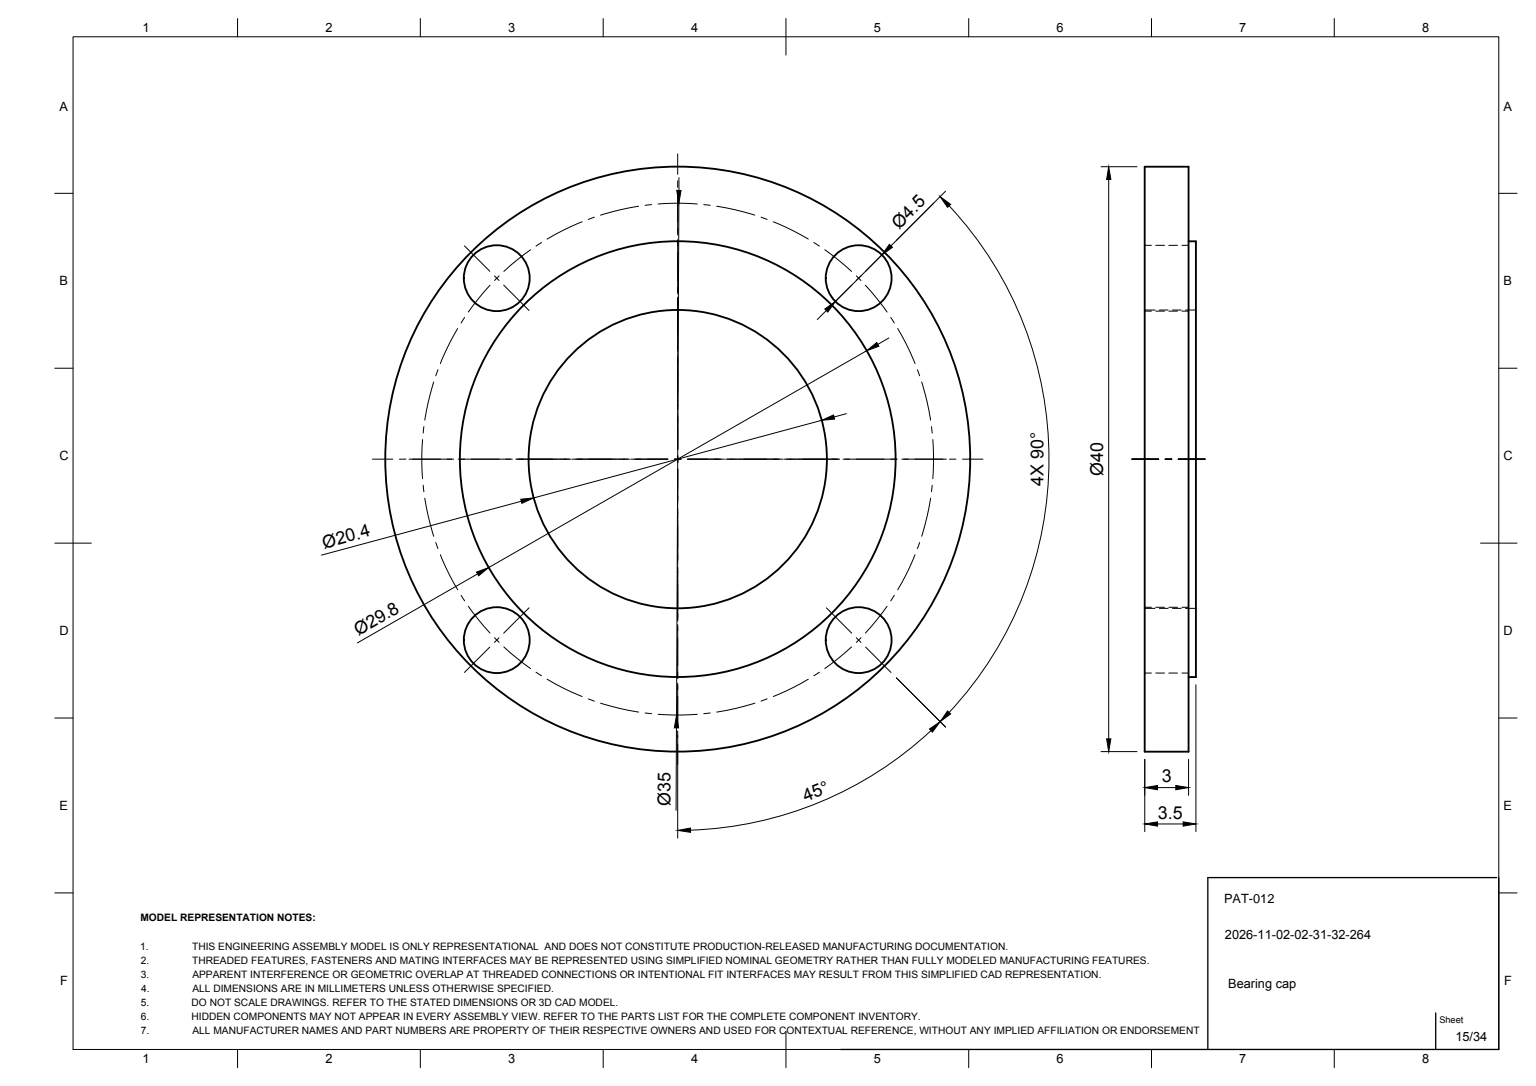
ISO-10303-21;
HEADER;
/* Generated by software containing ST-Developer
 * from STEP Tools, Inc. (www.steptools.com) 
 */

FILE_DESCRIPTION(
/* description */ ('Belt tensioner idler arm'),
/* implementation_level */ '2;1');

FILE_NAME(
/* name */ 'Bearing cap.step',
/* time_stamp */ '2026-10-28T03:22:15-07:00',
/* author */ (''),
/* organization */ (''),
/* preprocessor_version */ 'ST-DEVELOPER v20.2',
/* originating_system */ 'Autodesk Translation Framework v15.17.0.0',
/* authorisation */ '');

FILE_SCHEMA (('AUTOMOTIVE_DESIGN { 1 0 10303 214 3 1 1 }'));
ENDSEC;

DATA;
#10=MECHANICAL_DESIGN_GEOMETRIC_PRESENTATION_REPRESENTATION('',(#460),#12779);
#392=SHAPE_REPRESENTATION_RELATIONSHIP('SRR','None',#12939,#426);
#426=ADVANCED_BREP_SHAPE_REPRESENTATION('',(#500),#12756);
#460=STYLED_ITEM('',(#13184),#500);
#500=MANIFOLD_SOLID_BREP('Body1',#6196);
#582=FACE_BOUND('',#1400,.T.);
#583=FACE_BOUND('',#1404,.T.);
#584=FACE_BOUND('',#1405,.T.);
#585=FACE_BOUND('',#1406,.T.);
#586=FACE_BOUND('',#1407,.T.);
#587=FACE_BOUND('',#1408,.T.);
#588=FACE_BOUND('',#1410,.T.);
#589=FACE_BOUND('',#1411,.T.);
#590=FACE_BOUND('',#1412,.T.);
#591=FACE_BOUND('',#1413,.T.);
#592=FACE_BOUND('',#1414,.T.);
#744=PLANE('',#6866);
#745=PLANE('',#6873);
#746=PLANE('',#6874);
#972=FACE_OUTER_BOUND('',#1394,.T.);
#973=FACE_OUTER_BOUND('',#1395,.T.);
#974=FACE_OUTER_BOUND('',#1396,.T.);
#975=FACE_OUTER_BOUND('',#1397,.T.);
#976=FACE_OUTER_BOUND('',#1398,.T.);
#977=FACE_OUTER_BOUND('',#1399,.T.);
#978=FACE_OUTER_BOUND('',#1401,.T.);
#979=FACE_OUTER_BOUND('',#1402,.T.);
#980=FACE_OUTER_BOUND('',#1403,.T.);
#981=FACE_OUTER_BOUND('',#1409,.T.);
#1394=EDGE_LOOP('',(#4638,#4639,#4640,#4641));
#1395=EDGE_LOOP('',(#4642,#4643,#4644,#4645));
#1396=EDGE_LOOP('',(#4646,#4647,#4648,#4649));
#1397=EDGE_LOOP('',(#4650,#4651,#4652,#4653));
#1398=EDGE_LOOP('',(#4654,#4655,#4656,#4657));
#1399=EDGE_LOOP('',(#4658));
#1400=EDGE_LOOP('',(#4659));
#1401=EDGE_LOOP('',(#4660,#4661,#4662,#4663));
#1402=EDGE_LOOP('',(#4664,#4665,#4666,#4667));
#1403=EDGE_LOOP('',(#4668));
#1404=EDGE_LOOP('',(#4669));
#1405=EDGE_LOOP('',(#4670));
#1406=EDGE_LOOP('',(#4671));
#1407=EDGE_LOOP('',(#4672));
#1408=EDGE_LOOP('',(#4673));
#1409=EDGE_LOOP('',(#4674));
#1410=EDGE_LOOP('',(#4675));
#1411=EDGE_LOOP('',(#4676));
#1412=EDGE_LOOP('',(#4677));
#1413=EDGE_LOOP('',(#4678));
#1414=EDGE_LOOP('',(#4679));
#1861=LINE('',#10780,#2210);
#1862=LINE('',#10786,#2211);
#1863=LINE('',#10792,#2212);
#1864=LINE('',#10798,#2213);
#1865=LINE('',#10804,#2214);
#1866=LINE('',#10811,#2215);
#1867=LINE('',#10817,#2216);
#2210=VECTOR('',#8089,0.225);
#2211=VECTOR('',#8096,0.225);
#2212=VECTOR('',#8103,0.225);
#2213=VECTOR('',#8110,0.225);
#2214=VECTOR('',#8117,1.49);
#2215=VECTOR('',#8126,1.02);
#2216=VECTOR('',#8133,2.);
#2502=CIRCLE('',#6852,0.225);
#2503=CIRCLE('',#6853,0.225);
#2504=CIRCLE('',#6855,0.225);
#2505=CIRCLE('',#6856,0.225);
#2506=CIRCLE('',#6858,0.225);
#2507=CIRCLE('',#6859,0.225);
#2508=CIRCLE('',#6861,0.225);
#2509=CIRCLE('',#6862,0.225);
#2510=CIRCLE('',#6864,1.49);
#2511=CIRCLE('',#6865,1.49);
#2512=CIRCLE('',#6867,1.02);
#2513=CIRCLE('',#6869,1.02);
#2514=CIRCLE('',#6871,2.);
#2515=CIRCLE('',#6872,2.);
#2947=VERTEX_POINT('',#10777);
#2948=VERTEX_POINT('',#10779);
#2949=VERTEX_POINT('',#10783);
#2950=VERTEX_POINT('',#10785);
#2951=VERTEX_POINT('',#10789);
#2952=VERTEX_POINT('',#10791);
#2953=VERTEX_POINT('',#10795);
#2954=VERTEX_POINT('',#10797);
#2955=VERTEX_POINT('',#10801);
#2956=VERTEX_POINT('',#10803);
#2957=VERTEX_POINT('',#10807);
#2958=VERTEX_POINT('',#10810);
#2959=VERTEX_POINT('',#10814);
#2960=VERTEX_POINT('',#10816);
#3574=EDGE_CURVE('',#2947,#2947,#2502,.T.);
#3575=EDGE_CURVE('',#2947,#2948,#1861,.T.);
#3576=EDGE_CURVE('',#2948,#2948,#2503,.T.);
#3577=EDGE_CURVE('',#2949,#2949,#2504,.T.);
#3578=EDGE_CURVE('',#2949,#2950,#1862,.T.);
#3579=EDGE_CURVE('',#2950,#2950,#2505,.T.);
#3580=EDGE_CURVE('',#2951,#2951,#2506,.T.);
#3581=EDGE_CURVE('',#2951,#2952,#1863,.T.);
#3582=EDGE_CURVE('',#2952,#2952,#2507,.T.);
#3583=EDGE_CURVE('',#2953,#2953,#2508,.T.);
#3584=EDGE_CURVE('',#2953,#2954,#1864,.T.);
#3585=EDGE_CURVE('',#2954,#2954,#2509,.T.);
#3586=EDGE_CURVE('',#2955,#2955,#2510,.T.);
#3587=EDGE_CURVE('',#2955,#2956,#1865,.T.);
#3588=EDGE_CURVE('',#2956,#2956,#2511,.T.);
#3589=EDGE_CURVE('',#2957,#2957,#2512,.T.);
#3590=EDGE_CURVE('',#2957,#2958,#1866,.T.);
#3591=EDGE_CURVE('',#2958,#2958,#2513,.T.);
#3592=EDGE_CURVE('',#2959,#2959,#2514,.T.);
#3593=EDGE_CURVE('',#2959,#2960,#1867,.T.);
#3594=EDGE_CURVE('',#2960,#2960,#2515,.T.);
#4638=ORIENTED_EDGE('',*,*,#3574,.F.);
#4639=ORIENTED_EDGE('',*,*,#3575,.T.);
#4640=ORIENTED_EDGE('',*,*,#3576,.F.);
#4641=ORIENTED_EDGE('',*,*,#3575,.F.);
#4642=ORIENTED_EDGE('',*,*,#3577,.F.);
#4643=ORIENTED_EDGE('',*,*,#3578,.T.);
#4644=ORIENTED_EDGE('',*,*,#3579,.F.);
#4645=ORIENTED_EDGE('',*,*,#3578,.F.);
#4646=ORIENTED_EDGE('',*,*,#3580,.F.);
#4647=ORIENTED_EDGE('',*,*,#3581,.T.);
#4648=ORIENTED_EDGE('',*,*,#3582,.F.);
#4649=ORIENTED_EDGE('',*,*,#3581,.F.);
#4650=ORIENTED_EDGE('',*,*,#3583,.F.);
#4651=ORIENTED_EDGE('',*,*,#3584,.T.);
#4652=ORIENTED_EDGE('',*,*,#3585,.F.);
#4653=ORIENTED_EDGE('',*,*,#3584,.F.);
#4654=ORIENTED_EDGE('',*,*,#3586,.F.);
#4655=ORIENTED_EDGE('',*,*,#3587,.T.);
#4656=ORIENTED_EDGE('',*,*,#3588,.F.);
#4657=ORIENTED_EDGE('',*,*,#3587,.F.);
#4658=ORIENTED_EDGE('',*,*,#3586,.T.);
#4659=ORIENTED_EDGE('',*,*,#3589,.T.);
#4660=ORIENTED_EDGE('',*,*,#3589,.F.);
#4661=ORIENTED_EDGE('',*,*,#3590,.T.);
#4662=ORIENTED_EDGE('',*,*,#3591,.T.);
#4663=ORIENTED_EDGE('',*,*,#3590,.F.);
#4664=ORIENTED_EDGE('',*,*,#3592,.F.);
#4665=ORIENTED_EDGE('',*,*,#3593,.T.);
#4666=ORIENTED_EDGE('',*,*,#3594,.T.);
#4667=ORIENTED_EDGE('',*,*,#3593,.F.);
#4668=ORIENTED_EDGE('',*,*,#3592,.T.);
#4669=ORIENTED_EDGE('',*,*,#3588,.T.);
#4670=ORIENTED_EDGE('',*,*,#3585,.T.);
#4671=ORIENTED_EDGE('',*,*,#3582,.T.);
#4672=ORIENTED_EDGE('',*,*,#3579,.T.);
#4673=ORIENTED_EDGE('',*,*,#3576,.T.);
#4674=ORIENTED_EDGE('',*,*,#3594,.F.);
#4675=ORIENTED_EDGE('',*,*,#3591,.F.);
#4676=ORIENTED_EDGE('',*,*,#3583,.T.);
#4677=ORIENTED_EDGE('',*,*,#3580,.T.);
#4678=ORIENTED_EDGE('',*,*,#3577,.T.);
#4679=ORIENTED_EDGE('',*,*,#3574,.T.);
#5704=CYLINDRICAL_SURFACE('',#6851,0.225);
#5705=CYLINDRICAL_SURFACE('',#6854,0.225);
#5706=CYLINDRICAL_SURFACE('',#6857,0.225);
#5707=CYLINDRICAL_SURFACE('',#6860,0.225);
#5708=CYLINDRICAL_SURFACE('',#6863,1.49);
#5709=CYLINDRICAL_SURFACE('',#6868,1.02);
#5710=CYLINDRICAL_SURFACE('',#6870,2.);
#5949=ADVANCED_FACE('',(#972),#5704,.F.);
#5950=ADVANCED_FACE('',(#973),#5705,.F.);
#5951=ADVANCED_FACE('',(#974),#5706,.F.);
#5952=ADVANCED_FACE('',(#975),#5707,.F.);
#5953=ADVANCED_FACE('',(#976),#5708,.T.);
#5954=ADVANCED_FACE('',(#977,#582),#744,.T.);
#5955=ADVANCED_FACE('',(#978),#5709,.F.);
#5956=ADVANCED_FACE('',(#979),#5710,.T.);
#5957=ADVANCED_FACE('',(#980,#583,#584,#585,#586,#587),#745,.T.);
#5958=ADVANCED_FACE('',(#981,#588,#589,#590,#591,#592),#746,.F.);
#6196=CLOSED_SHELL('',(#5949,#5950,#5951,#5952,#5953,#5954,#5955,#5956,
#5957,#5958));
#6850=AXIS2_PLACEMENT_3D('',#10775,#8083,#8084);
#6851=AXIS2_PLACEMENT_3D('',#10776,#8085,#8086);
#6852=AXIS2_PLACEMENT_3D('',#10778,#8087,#8088);
#6853=AXIS2_PLACEMENT_3D('',#10781,#8090,#8091);
#6854=AXIS2_PLACEMENT_3D('',#10782,#8092,#8093);
#6855=AXIS2_PLACEMENT_3D('',#10784,#8094,#8095);
#6856=AXIS2_PLACEMENT_3D('',#10787,#8097,#8098);
#6857=AXIS2_PLACEMENT_3D('',#10788,#8099,#8100);
#6858=AXIS2_PLACEMENT_3D('',#10790,#8101,#8102);
#6859=AXIS2_PLACEMENT_3D('',#10793,#8104,#8105);
#6860=AXIS2_PLACEMENT_3D('',#10794,#8106,#8107);
#6861=AXIS2_PLACEMENT_3D('',#10796,#8108,#8109);
#6862=AXIS2_PLACEMENT_3D('',#10799,#8111,#8112);
#6863=AXIS2_PLACEMENT_3D('',#10800,#8113,#8114);
#6864=AXIS2_PLACEMENT_3D('',#10802,#8115,#8116);
#6865=AXIS2_PLACEMENT_3D('',#10805,#8118,#8119);
#6866=AXIS2_PLACEMENT_3D('',#10806,#8120,#8121);
#6867=AXIS2_PLACEMENT_3D('',#10808,#8122,#8123);
#6868=AXIS2_PLACEMENT_3D('',#10809,#8124,#8125);
#6869=AXIS2_PLACEMENT_3D('',#10812,#8127,#8128);
#6870=AXIS2_PLACEMENT_3D('',#10813,#8129,#8130);
#6871=AXIS2_PLACEMENT_3D('',#10815,#8131,#8132);
#6872=AXIS2_PLACEMENT_3D('',#10818,#8134,#8135);
#6873=AXIS2_PLACEMENT_3D('',#10819,#8136,#8137);
#6874=AXIS2_PLACEMENT_3D('',#10820,#8138,#8139);
#8083=DIRECTION('axis',(0.,0.,1.));
#8084=DIRECTION('refdir',(1.,0.,0.));
#8085=DIRECTION('center_axis',(0.,0.,1.));
#8086=DIRECTION('ref_axis',(1.,0.,0.));
#8087=DIRECTION('center_axis',(0.,0.,1.));
#8088=DIRECTION('ref_axis',(1.,0.,0.));
#8089=DIRECTION('',(0.,0.,1.));
#8090=DIRECTION('center_axis',(0.,0.,-1.));
#8091=DIRECTION('ref_axis',(1.,0.,0.));
#8092=DIRECTION('center_axis',(0.,0.,1.));
#8093=DIRECTION('ref_axis',(1.,0.,0.));
#8094=DIRECTION('center_axis',(0.,0.,1.));
#8095=DIRECTION('ref_axis',(1.,0.,0.));
#8096=DIRECTION('',(0.,0.,1.));
#8097=DIRECTION('center_axis',(0.,0.,-1.));
#8098=DIRECTION('ref_axis',(1.,0.,0.));
#8099=DIRECTION('center_axis',(0.,0.,1.));
#8100=DIRECTION('ref_axis',(1.,0.,0.));
#8101=DIRECTION('center_axis',(0.,0.,1.));
#8102=DIRECTION('ref_axis',(1.,0.,0.));
#8103=DIRECTION('',(0.,0.,1.));
#8104=DIRECTION('center_axis',(0.,0.,-1.));
#8105=DIRECTION('ref_axis',(1.,0.,0.));
#8106=DIRECTION('center_axis',(0.,0.,1.));
#8107=DIRECTION('ref_axis',(1.,0.,0.));
#8108=DIRECTION('center_axis',(0.,0.,1.));
#8109=DIRECTION('ref_axis',(1.,0.,0.));
#8110=DIRECTION('',(0.,0.,1.));
#8111=DIRECTION('center_axis',(0.,0.,-1.));
#8112=DIRECTION('ref_axis',(1.,0.,0.));
#8113=DIRECTION('center_axis',(0.,0.,1.));
#8114=DIRECTION('ref_axis',(1.,0.,0.));
#8115=DIRECTION('center_axis',(0.,0.,1.));
#8116=DIRECTION('ref_axis',(1.,0.,0.));
#8117=DIRECTION('',(0.,0.,-1.));
#8118=DIRECTION('center_axis',(0.,0.,-1.));
#8119=DIRECTION('ref_axis',(1.,0.,0.));
#8120=DIRECTION('center_axis',(0.,0.,1.));
#8121=DIRECTION('ref_axis',(1.,0.,0.));
#8122=DIRECTION('center_axis',(0.,0.,-1.));
#8123=DIRECTION('ref_axis',(1.,0.,0.));
#8124=DIRECTION('center_axis',(0.,0.,1.));
#8125=DIRECTION('ref_axis',(1.,0.,0.));
#8126=DIRECTION('',(0.,0.,-1.));
#8127=DIRECTION('center_axis',(0.,0.,-1.));
#8128=DIRECTION('ref_axis',(1.,0.,0.));
#8129=DIRECTION('center_axis',(0.,0.,1.));
#8130=DIRECTION('ref_axis',(1.,0.,0.));
#8131=DIRECTION('center_axis',(0.,0.,1.));
#8132=DIRECTION('ref_axis',(1.,0.,0.));
#8133=DIRECTION('',(0.,0.,-1.));
#8134=DIRECTION('center_axis',(0.,0.,1.));
#8135=DIRECTION('ref_axis',(1.,0.,0.));
#8136=DIRECTION('center_axis',(0.,0.,1.));
#8137=DIRECTION('ref_axis',(1.,0.,0.));
#8138=DIRECTION('center_axis',(0.,0.,1.));
#8139=DIRECTION('ref_axis',(1.,0.,0.));
#10775=CARTESIAN_POINT('',(0.,0.,0.));
#10776=CARTESIAN_POINT('Origin',(-1.23743686707646,-1.23743686707646,4.6));
#10777=CARTESIAN_POINT('',(-1.46243686707646,-1.23743686707646,4.7));
#10778=CARTESIAN_POINT('Origin',(-1.23743686707646,-1.23743686707646,4.7));
#10779=CARTESIAN_POINT('',(-1.46243686707646,-1.23743686707646,5.));
#10780=CARTESIAN_POINT('',(-1.46243686707646,-1.23743686707646,4.6));
#10781=CARTESIAN_POINT('Origin',(-1.23743686707646,-1.23743686707646,5.));
#10782=CARTESIAN_POINT('Origin',(-1.23743686707646,1.23743686707646,4.6));
#10783=CARTESIAN_POINT('',(-1.46243686707646,1.23743686707646,4.7));
#10784=CARTESIAN_POINT('Origin',(-1.23743686707646,1.23743686707646,4.7));
#10785=CARTESIAN_POINT('',(-1.46243686707646,1.23743686707646,5.));
#10786=CARTESIAN_POINT('',(-1.46243686707646,1.23743686707646,4.6));
#10787=CARTESIAN_POINT('Origin',(-1.23743686707646,1.23743686707646,5.));
#10788=CARTESIAN_POINT('Origin',(1.23743686707646,1.23743686707646,4.6));
#10789=CARTESIAN_POINT('',(1.01243686707646,1.23743686707646,4.7));
#10790=CARTESIAN_POINT('Origin',(1.23743686707646,1.23743686707646,4.7));
#10791=CARTESIAN_POINT('',(1.01243686707646,1.23743686707646,5.));
#10792=CARTESIAN_POINT('',(1.01243686707646,1.23743686707646,4.6));
#10793=CARTESIAN_POINT('Origin',(1.23743686707646,1.23743686707646,5.));
#10794=CARTESIAN_POINT('Origin',(1.23743686707646,-1.23743686707646,4.6));
#10795=CARTESIAN_POINT('',(1.01243686707646,-1.23743686707646,4.7));
#10796=CARTESIAN_POINT('Origin',(1.23743686707646,-1.23743686707646,4.7));
#10797=CARTESIAN_POINT('',(1.01243686707646,-1.23743686707646,5.));
#10798=CARTESIAN_POINT('',(1.01243686707646,-1.23743686707646,4.6));
#10799=CARTESIAN_POINT('Origin',(1.23743686707646,-1.23743686707646,5.));
#10800=CARTESIAN_POINT('Origin',(0.,0.,5.));
#10801=CARTESIAN_POINT('',(-1.49,-1.82472373072956E-16,5.05));
#10802=CARTESIAN_POINT('Origin',(0.,0.,5.05));
#10803=CARTESIAN_POINT('',(-1.49,-1.82472373072956E-16,5.));
#10804=CARTESIAN_POINT('',(-1.49,-1.82472373072956E-16,5.));
#10805=CARTESIAN_POINT('Origin',(0.,0.,5.));
#10806=CARTESIAN_POINT('Origin',(0.,0.,5.05));
#10807=CARTESIAN_POINT('',(-1.02,-1.2491397351303E-16,5.05));
#10808=CARTESIAN_POINT('Origin',(0.,0.,5.05));
#10809=CARTESIAN_POINT('Origin',(0.,0.,4.7));
#10810=CARTESIAN_POINT('',(-1.02,-1.2491397351303E-16,4.7));
#10811=CARTESIAN_POINT('',(-1.02,-1.2491397351303E-16,4.7));
#10812=CARTESIAN_POINT('Origin',(0.,0.,4.7));
#10813=CARTESIAN_POINT('Origin',(0.,0.,4.7));
#10814=CARTESIAN_POINT('',(-2.,-2.44929359829471E-16,5.));
#10815=CARTESIAN_POINT('Origin',(0.,0.,5.));
#10816=CARTESIAN_POINT('',(-2.,-2.44929359829471E-16,4.7));
#10817=CARTESIAN_POINT('',(-2.,-2.44929359829471E-16,4.7));
#10818=CARTESIAN_POINT('Origin',(0.,0.,4.7));
#10819=CARTESIAN_POINT('Origin',(0.,0.,5.));
#10820=CARTESIAN_POINT('Origin',(0.,0.,4.7));
#12716=UNCERTAINTY_MEASURE_WITH_UNIT(LENGTH_MEASURE(0.001),#12780,
'DISTANCE_ACCURACY_VALUE',
'Maximum model space distance between geometric entities at asserted c
onnectivities');
#12739=UNCERTAINTY_MEASURE_WITH_UNIT(LENGTH_MEASURE(0.001),#12780,
'DISTANCE_ACCURACY_VALUE',
'Maximum model space distance between geometric entities at asserted c
onnectivities');
#12756=(
GEOMETRIC_REPRESENTATION_CONTEXT(3)
GLOBAL_UNCERTAINTY_ASSIGNED_CONTEXT((#12716))
GLOBAL_UNIT_ASSIGNED_CONTEXT((#12780,#12782,#12783))
REPRESENTATION_CONTEXT('','3D')
);
#12779=(
GEOMETRIC_REPRESENTATION_CONTEXT(3)
GLOBAL_UNCERTAINTY_ASSIGNED_CONTEXT((#12739))
GLOBAL_UNIT_ASSIGNED_CONTEXT((#12780,#12782,#12783))
REPRESENTATION_CONTEXT('','3D')
);
#12780=(
LENGTH_UNIT()
NAMED_UNIT(*)
SI_UNIT(.CENTI.,.METRE.)
);
#12782=(
NAMED_UNIT(*)
PLANE_ANGLE_UNIT()
SI_UNIT($,.RADIAN.)
);
#12783=(
NAMED_UNIT(*)
SI_UNIT($,.STERADIAN.)
SOLID_ANGLE_UNIT()
);
#12800=SHAPE_DEFINITION_REPRESENTATION(#12839,#12939);
#12839=PRODUCT_DEFINITION_SHAPE('',$,#12979);
#12939=SHAPE_REPRESENTATION('',(#6850),#12756);
#12962=PRODUCT_DEFINITION_CONTEXT('part definition',#13081,'design');
#12979=PRODUCT_DEFINITION('Bearing cap','Bearing cap',#13018,#12962);
#13018=PRODUCT_DEFINITION_FORMATION('',$,#13099);
#13081=APPLICATION_CONTEXT(
'Core Data for Automotive Mechanical Design Process');
#13082=PRODUCT_CONTEXT('part definition',#13081,'mechanical');
#13099=PRODUCT('Bearing cap','Bearing cap','Bearing cap',(#13082));
#13178=COLOUR_RGB('Grey',0.48,0.52,0.57);
#13179=FILL_AREA_STYLE_COLOUR('',#13178);
#13180=FILL_AREA_STYLE('',(#13179));
#13181=SURFACE_STYLE_FILL_AREA(#13180);
#13182=SURFACE_SIDE_STYLE('',(#13181));
#13183=SURFACE_STYLE_USAGE(.BOTH.,#13182);
#13184=PRESENTATION_STYLE_ASSIGNMENT((#13183));
ENDSEC;
END-ISO-10303-21;
